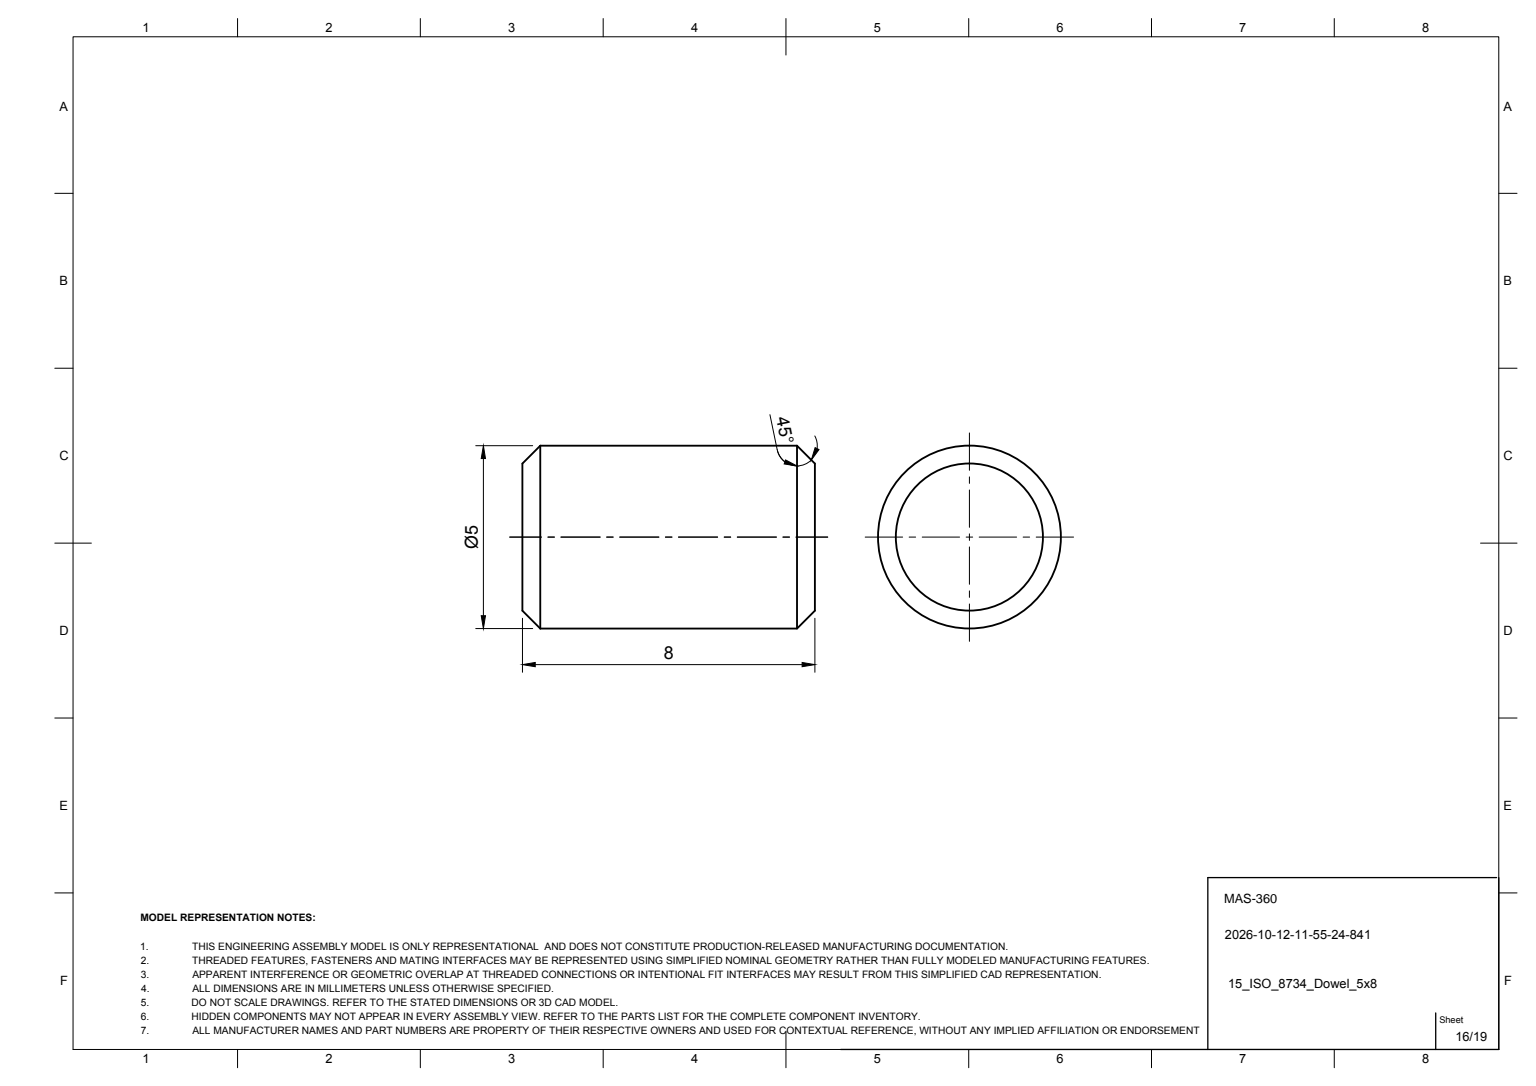
ISO-10303-21;
HEADER;
/* Generated by software containing ST-Developer
 * from STEP Tools, Inc. (www.steptools.com) 
 */

FILE_DESCRIPTION(
/* description */ (''),
/* implementation_level */ '2;1');

FILE_NAME(
/* name */ '15_ISO_8734_Dowel_5x8.step',
/* time_stamp */ '2026-11-04T18:53:29-08:00',
/* author */ (''),
/* organization */ (''),
/* preprocessor_version */ 'ST-DEVELOPER v20.2',
/* originating_system */ 'Autodesk Translation Framework v15.17.0.0',
/* authorisation */ '');

FILE_SCHEMA (('AUTOMOTIVE_DESIGN { 1 0 10303 214 3 1 1 }'));
ENDSEC;

DATA;
#10=MECHANICAL_DESIGN_GEOMETRIC_PRESENTATION_REPRESENTATION('',(#1342),#100031);
#246=CONICAL_SURFACE('',#22466,2.2552,0.785398163397448);
#247=CONICAL_SURFACE('',#22471,2.2552,0.785398163397448);
#1169=CIRCLE('',#22467,2.5);
#1170=CIRCLE('',#22468,2.0104);
#1171=CIRCLE('',#22470,2.5);
#1172=CIRCLE('',#22472,2.0104);
#1306=SHAPE_REPRESENTATION_RELATIONSHIP('SRR','None',#100116,#1324);
#1324=ADVANCED_BREP_SHAPE_REPRESENTATION('',(#1360),#100028);
#1342=STYLED_ITEM('',(#100204),#1360);
#1360=MANIFOLD_SOLID_BREP('Body1',#20132);
#1687=PLANE('',#22473);
#1688=PLANE('',#22474);
#3259=LINE('',#99915,#4546);
#3260=LINE('',#99920,#4547);
#3261=LINE('',#99923,#4548);
#4546=VECTOR('',#28072,2.2552);
#4547=VECTOR('',#28079,2.5);
#4548=VECTOR('',#28082,2.2552);
#5022=CYLINDRICAL_SURFACE('',#22469,2.5);
#6166=FACE_OUTER_BOUND('',#7437,.T.);
#6167=FACE_OUTER_BOUND('',#7438,.T.);
#6168=FACE_OUTER_BOUND('',#7439,.T.);
#6169=FACE_OUTER_BOUND('',#7440,.T.);
#6170=FACE_OUTER_BOUND('',#7441,.T.);
#7437=EDGE_LOOP('',(#18805,#18806,#18807,#18808));
#7438=EDGE_LOOP('',(#18809,#18810,#18811,#18812));
#7439=EDGE_LOOP('',(#18813,#18814,#18815,#18816));
#7440=EDGE_LOOP('',(#18817));
#7441=EDGE_LOOP('',(#18818));
#9910=VERTEX_POINT('',#99912);
#9911=VERTEX_POINT('',#99914);
#9912=VERTEX_POINT('',#99918);
#9913=VERTEX_POINT('',#99922);
#12877=EDGE_CURVE('',#9910,#9910,#1169,.T.);
#12878=EDGE_CURVE('',#9910,#9911,#3259,.T.);
#12879=EDGE_CURVE('',#9911,#9911,#1170,.T.);
#12880=EDGE_CURVE('',#9912,#9912,#1171,.T.);
#12881=EDGE_CURVE('',#9912,#9910,#3260,.T.);
#12882=EDGE_CURVE('',#9912,#9913,#3261,.T.);
#12883=EDGE_CURVE('',#9913,#9913,#1172,.T.);
#18805=ORIENTED_EDGE('',*,*,#12877,.F.);
#18806=ORIENTED_EDGE('',*,*,#12878,.T.);
#18807=ORIENTED_EDGE('',*,*,#12879,.T.);
#18808=ORIENTED_EDGE('',*,*,#12878,.F.);
#18809=ORIENTED_EDGE('',*,*,#12880,.F.);
#18810=ORIENTED_EDGE('',*,*,#12881,.T.);
#18811=ORIENTED_EDGE('',*,*,#12877,.T.);
#18812=ORIENTED_EDGE('',*,*,#12881,.F.);
#18813=ORIENTED_EDGE('',*,*,#12880,.T.);
#18814=ORIENTED_EDGE('',*,*,#12882,.T.);
#18815=ORIENTED_EDGE('',*,*,#12883,.F.);
#18816=ORIENTED_EDGE('',*,*,#12882,.F.);
#18817=ORIENTED_EDGE('',*,*,#12883,.T.);
#18818=ORIENTED_EDGE('',*,*,#12879,.F.);
#20100=ADVANCED_FACE('',(#6166),#246,.T.);
#20101=ADVANCED_FACE('',(#6167),#5022,.T.);
#20102=ADVANCED_FACE('',(#6168),#247,.T.);
#20103=ADVANCED_FACE('',(#6169),#1687,.T.);
#20104=ADVANCED_FACE('',(#6170),#1688,.T.);
#20132=CLOSED_SHELL('',(#20100,#20101,#20102,#20103,#20104));
#22465=AXIS2_PLACEMENT_3D('',#99910,#28066,#28067);
#22466=AXIS2_PLACEMENT_3D('',#99911,#28068,#28069);
#22467=AXIS2_PLACEMENT_3D('',#99913,#28070,#28071);
#22468=AXIS2_PLACEMENT_3D('',#99916,#28073,#28074);
#22469=AXIS2_PLACEMENT_3D('',#99917,#28075,#28076);
#22470=AXIS2_PLACEMENT_3D('',#99919,#28077,#28078);
#22471=AXIS2_PLACEMENT_3D('',#99921,#28080,#28081);
#22472=AXIS2_PLACEMENT_3D('',#99924,#28083,#28084);
#22473=AXIS2_PLACEMENT_3D('',#99925,#28085,#28086);
#22474=AXIS2_PLACEMENT_3D('',#99926,#28087,#28088);
#28066=DIRECTION('axis',(0.,0.,1.));
#28067=DIRECTION('refdir',(1.,0.,0.));
#28068=DIRECTION('center_axis',(1.,0.,0.));
#28069=DIRECTION('ref_axis',(0.,1.,0.));
#28070=DIRECTION('center_axis',(1.,0.,0.));
#28071=DIRECTION('ref_axis',(0.,0.,-1.));
#28072=DIRECTION('',(-0.707106781186548,0.707106781186547,8.65956056235493E-17));
#28073=DIRECTION('center_axis',(1.,0.,0.));
#28074=DIRECTION('ref_axis',(0.,0.,-1.));
#28075=DIRECTION('center_axis',(1.,0.,0.));
#28076=DIRECTION('ref_axis',(0.,1.,0.));
#28077=DIRECTION('center_axis',(1.,0.,0.));
#28078=DIRECTION('ref_axis',(0.,0.,-1.));
#28079=DIRECTION('',(-1.,0.,0.));
#28080=DIRECTION('center_axis',(-1.,0.,0.));
#28081=DIRECTION('ref_axis',(0.,1.,0.));
#28082=DIRECTION('',(0.707106781186548,0.707106781186547,-8.65956056235493E-17));
#28083=DIRECTION('center_axis',(1.,0.,0.));
#28084=DIRECTION('ref_axis',(0.,0.,-1.));
#28085=DIRECTION('center_axis',(1.,0.,0.));
#28086=DIRECTION('ref_axis',(0.,0.,-1.));
#28087=DIRECTION('center_axis',(-1.,0.,0.));
#28088=DIRECTION('ref_axis',(0.,0.,1.));
#99910=CARTESIAN_POINT('',(0.,0.,0.));
#99911=CARTESIAN_POINT('Origin',(0.2448,0.,0.));
#99912=CARTESIAN_POINT('',(0.4896,-2.5,-3.06161699786838E-16));
#99913=CARTESIAN_POINT('Origin',(0.4896,0.,0.));
#99914=CARTESIAN_POINT('',(0.,-2.0104,-2.46202992500584E-16));
#99915=CARTESIAN_POINT('',(0.2448,-2.2552,-2.76182346143711E-16));
#99916=CARTESIAN_POINT('Origin',(0.,0.,0.));
#99917=CARTESIAN_POINT('Origin',(4.,0.,0.));
#99918=CARTESIAN_POINT('',(7.5104,-2.5,-3.06161699786838E-16));
#99919=CARTESIAN_POINT('Origin',(7.5104,0.,0.));
#99920=CARTESIAN_POINT('',(4.,-2.5,-3.06161699786838E-16));
#99921=CARTESIAN_POINT('Origin',(7.7552,0.,0.));
#99922=CARTESIAN_POINT('',(8.,-2.0104,-2.46202992500584E-16));
#99923=CARTESIAN_POINT('',(7.7552,-2.2552,2.76182346143711E-16));
#99924=CARTESIAN_POINT('Origin',(8.,0.,0.));
#99925=CARTESIAN_POINT('Origin',(8.,0.,0.));
#99926=CARTESIAN_POINT('Origin',(0.,2.0104,0.));
#100008=UNCERTAINTY_MEASURE_WITH_UNIT(LENGTH_MEASURE(0.01),#100032,
'DISTANCE_ACCURACY_VALUE',
'Maximum model space distance between geometric entities at asserted c
onnectivities');
#100011=UNCERTAINTY_MEASURE_WITH_UNIT(LENGTH_MEASURE(0.01),#100032,
'DISTANCE_ACCURACY_VALUE',
'Maximum model space distance between geometric entities at asserted c
onnectivities');
#100028=(
GEOMETRIC_REPRESENTATION_CONTEXT(3)
GLOBAL_UNCERTAINTY_ASSIGNED_CONTEXT((#100008))
GLOBAL_UNIT_ASSIGNED_CONTEXT((#100032,#100034,#100035))
REPRESENTATION_CONTEXT('','3D')
);
#100031=(
GEOMETRIC_REPRESENTATION_CONTEXT(3)
GLOBAL_UNCERTAINTY_ASSIGNED_CONTEXT((#100011))
GLOBAL_UNIT_ASSIGNED_CONTEXT((#100032,#100034,#100035))
REPRESENTATION_CONTEXT('','3D')
);
#100032=(
LENGTH_UNIT()
NAMED_UNIT(*)
SI_UNIT(.MILLI.,.METRE.)
);
#100034=(
NAMED_UNIT(*)
PLANE_ANGLE_UNIT()
SI_UNIT($,.RADIAN.)
);
#100035=(
NAMED_UNIT(*)
SI_UNIT($,.STERADIAN.)
SOLID_ANGLE_UNIT()
);
#100052=SHAPE_DEFINITION_REPRESENTATION(#100071,#100116);
#100071=PRODUCT_DEFINITION_SHAPE('',$,#100136);
#100116=SHAPE_REPRESENTATION('',(#22465),#100028);
#100119=PRODUCT_DEFINITION_CONTEXT('part definition',#100178,'design');
#100136=PRODUCT_DEFINITION('2026-10-12-11-55-24-841',
'15_ISO_8734_Dowel_5x8',#100155,#100119);
#100155=PRODUCT_DEFINITION_FORMATION('',$,#100196);
#100178=APPLICATION_CONTEXT(
'Core Data for Automotive Mechanical Design Process');
#100179=PRODUCT_CONTEXT('part definition',#100178,'mechanical');
#100196=PRODUCT('2026-10-12-11-55-24-841','15_ISO_8734_Dowel_5x8',$,(#100179));
#100204=PRESENTATION_STYLE_ASSIGNMENT((#100210));
#100210=SURFACE_STYLE_USAGE(.BOTH.,#100216);
#100216=SURFACE_SIDE_STYLE('',(#100222));
#100222=SURFACE_STYLE_FILL_AREA(#100228);
#100228=FILL_AREA_STYLE('Opaque(97,158,199)',(#100234));
#100234=FILL_AREA_STYLE_COLOUR('Opaque(97,158,199)',#100240);
#100240=COLOUR_RGB('Opaque(97,158,199)',0.380392156862745,0.619607843137255,
0.780392156862745);
ENDSEC;
END-ISO-10303-21;
